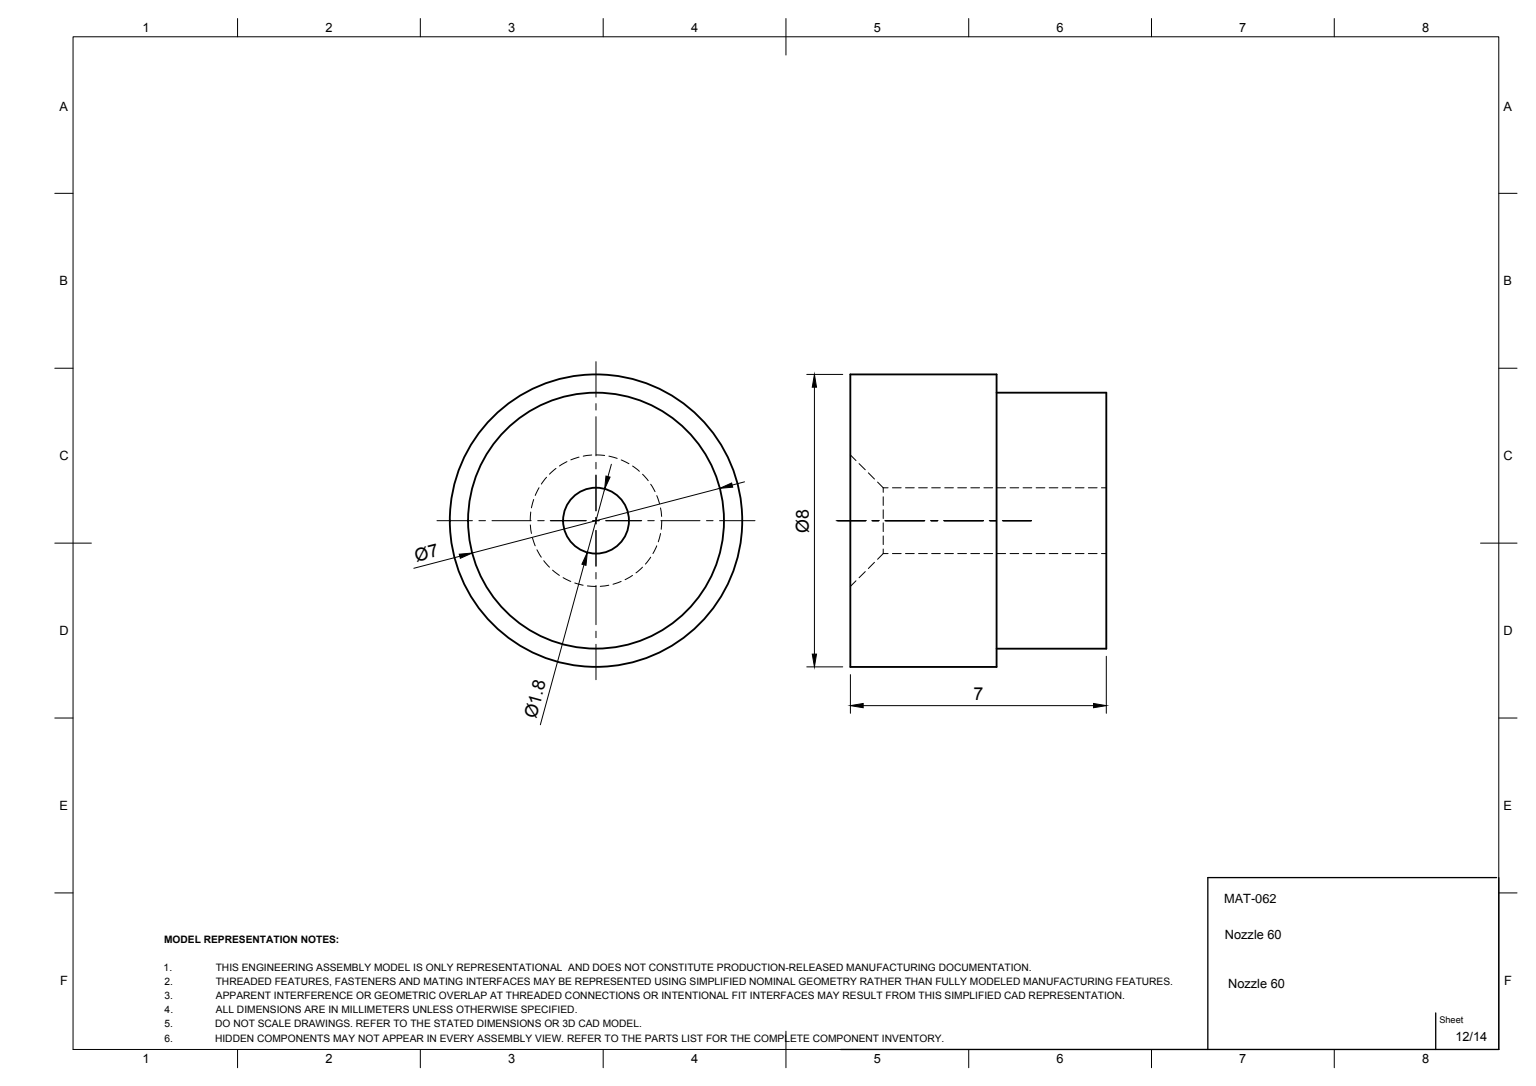
ISO-10303-21;
HEADER;
/* Generated by software containing ST-Developer
 * from STEP Tools, Inc. (www.steptools.com) 
 */

FILE_DESCRIPTION(
/* description */ (''),
/* implementation_level */ '2;1');

FILE_NAME(
/* name */ 'Nozzle 60.step',
/* time_stamp */ '2026-10-24T10:18:25-07:00',
/* author */ (''),
/* organization */ (''),
/* preprocessor_version */ 'ST-DEVELOPER v20.2',
/* originating_system */ 'Autodesk Translation Framework v15.15.0.0',
/* authorisation */ '');

FILE_SCHEMA (('AUTOMOTIVE_DESIGN { 1 0 10303 214 3 1 1 }'));
ENDSEC;

DATA;
#10=MECHANICAL_DESIGN_GEOMETRIC_PRESENTATION_REPRESENTATION('',(#260),#14125);
#194=CONICAL_SURFACE('',#6620,1.8,0.785398163397439);
#231=SHAPE_REPRESENTATION_RELATIONSHIP('SRR','None',#14205,#241);
#241=ADVANCED_BREP_SHAPE_REPRESENTATION('',(#273),#14119);
#260=STYLED_ITEM('',(#14263),#273);
#273=MANIFOLD_SOLID_BREP('Nozzle 60',#6141);
#554=CYLINDRICAL_SURFACE('',#6610,3.99999999999999);
#555=CYLINDRICAL_SURFACE('',#6617,0.899999999999993);
#556=CYLINDRICAL_SURFACE('',#6623,3.49999999999999);
#675=FACE_BOUND('',#1342,.T.);
#676=FACE_BOUND('',#1344,.T.);
#677=FACE_BOUND('',#1348,.T.);
#939=FACE_OUTER_BOUND('',#1340,.T.);
#940=FACE_OUTER_BOUND('',#1341,.T.);
#941=FACE_OUTER_BOUND('',#1343,.T.);
#942=FACE_OUTER_BOUND('',#1345,.T.);
#943=FACE_OUTER_BOUND('',#1346,.T.);
#944=FACE_OUTER_BOUND('',#1347,.T.);
#945=FACE_OUTER_BOUND('',#1349,.T.);
#1340=EDGE_LOOP('',(#4981,#4982,#4983,#4984));
#1341=EDGE_LOOP('',(#4985));
#1342=EDGE_LOOP('',(#4986));
#1343=EDGE_LOOP('',(#4987));
#1344=EDGE_LOOP('',(#4988));
#1345=EDGE_LOOP('',(#4989,#4990,#4991,#4992));
#1346=EDGE_LOOP('',(#4993,#4994,#4995,#4996));
#1347=EDGE_LOOP('',(#4997));
#1348=EDGE_LOOP('',(#4998));
#1349=EDGE_LOOP('',(#4999,#5000,#5001,#5002));
#1699=CIRCLE('',#6611,3.99999999999999);
#1700=CIRCLE('',#6612,3.99999999999999);
#1701=CIRCLE('',#6614,3.49999999999999);
#1702=CIRCLE('',#6616,1.8);
#1703=CIRCLE('',#6618,0.899999999999989);
#1704=CIRCLE('',#6619,0.899999999999988);
#1705=CIRCLE('',#6622,3.49999999999999);
#2038=LINE('',#12218,#2426);
#2039=LINE('',#12230,#2427);
#2040=LINE('',#12233,#2428);
#2041=LINE('',#12238,#2429);
#2426=VECTOR('',#7850,3.99999999999999);
#2427=VECTOR('',#7865,0.899999999999994);
#2428=VECTOR('',#7870,1.8);
#2429=VECTOR('',#7877,3.49999999999999);
#2916=VERTEX_POINT('',#12215);
#2917=VERTEX_POINT('',#12217);
#2918=VERTEX_POINT('',#12221);
#2919=VERTEX_POINT('',#12224);
#2920=VERTEX_POINT('',#12227);
#2921=VERTEX_POINT('',#12229);
#2922=VERTEX_POINT('',#12235);
#3638=EDGE_CURVE('',#2916,#2916,#1699,.T.);
#3639=EDGE_CURVE('',#2916,#2917,#2038,.T.);
#3640=EDGE_CURVE('',#2917,#2917,#1700,.T.);
#3641=EDGE_CURVE('',#2918,#2918,#1701,.T.);
#3642=EDGE_CURVE('',#2919,#2919,#1702,.T.);
#3643=EDGE_CURVE('',#2920,#2920,#1703,.T.);
#3644=EDGE_CURVE('',#2920,#2921,#2039,.T.);
#3645=EDGE_CURVE('',#2921,#2921,#1704,.T.);
#3646=EDGE_CURVE('',#2921,#2919,#2040,.T.);
#3647=EDGE_CURVE('',#2922,#2922,#1705,.T.);
#3648=EDGE_CURVE('',#2918,#2922,#2041,.T.);
#4981=ORIENTED_EDGE('',*,*,#3638,.T.);
#4982=ORIENTED_EDGE('',*,*,#3639,.T.);
#4983=ORIENTED_EDGE('',*,*,#3640,.F.);
#4984=ORIENTED_EDGE('',*,*,#3639,.F.);
#4985=ORIENTED_EDGE('',*,*,#3640,.T.);
#4986=ORIENTED_EDGE('',*,*,#3641,.F.);
#4987=ORIENTED_EDGE('',*,*,#3638,.F.);
#4988=ORIENTED_EDGE('',*,*,#3642,.F.);
#4989=ORIENTED_EDGE('',*,*,#3643,.T.);
#4990=ORIENTED_EDGE('',*,*,#3644,.T.);
#4991=ORIENTED_EDGE('',*,*,#3645,.T.);
#4992=ORIENTED_EDGE('',*,*,#3644,.F.);
#4993=ORIENTED_EDGE('',*,*,#3645,.F.);
#4994=ORIENTED_EDGE('',*,*,#3646,.T.);
#4995=ORIENTED_EDGE('',*,*,#3642,.T.);
#4996=ORIENTED_EDGE('',*,*,#3646,.F.);
#4997=ORIENTED_EDGE('',*,*,#3647,.T.);
#4998=ORIENTED_EDGE('',*,*,#3643,.F.);
#4999=ORIENTED_EDGE('',*,*,#3641,.T.);
#5000=ORIENTED_EDGE('',*,*,#3648,.T.);
#5001=ORIENTED_EDGE('',*,*,#3647,.F.);
#5002=ORIENTED_EDGE('',*,*,#3648,.F.);
#5716=PLANE('',#6613);
#5717=PLANE('',#6615);
#5718=PLANE('',#6621);
#5988=ADVANCED_FACE('',(#939),#554,.T.);
#5989=ADVANCED_FACE('',(#940,#675),#5716,.T.);
#5990=ADVANCED_FACE('',(#941,#676),#5717,.F.);
#5991=ADVANCED_FACE('',(#942),#555,.F.);
#5992=ADVANCED_FACE('',(#943),#194,.F.);
#5993=ADVANCED_FACE('',(#944,#677),#5718,.T.);
#5994=ADVANCED_FACE('',(#945),#556,.T.);
#6141=CLOSED_SHELL('',(#5988,#5989,#5990,#5991,#5992,#5993,#5994));
#6609=AXIS2_PLACEMENT_3D('',#12213,#7844,#7845);
#6610=AXIS2_PLACEMENT_3D('',#12214,#7846,#7847);
#6611=AXIS2_PLACEMENT_3D('',#12216,#7848,#7849);
#6612=AXIS2_PLACEMENT_3D('',#12219,#7851,#7852);
#6613=AXIS2_PLACEMENT_3D('',#12220,#7853,#7854);
#6614=AXIS2_PLACEMENT_3D('',#12222,#7855,#7856);
#6615=AXIS2_PLACEMENT_3D('',#12223,#7857,#7858);
#6616=AXIS2_PLACEMENT_3D('',#12225,#7859,#7860);
#6617=AXIS2_PLACEMENT_3D('',#12226,#7861,#7862);
#6618=AXIS2_PLACEMENT_3D('',#12228,#7863,#7864);
#6619=AXIS2_PLACEMENT_3D('',#12231,#7866,#7867);
#6620=AXIS2_PLACEMENT_3D('',#12232,#7868,#7869);
#6621=AXIS2_PLACEMENT_3D('',#12234,#7871,#7872);
#6622=AXIS2_PLACEMENT_3D('',#12236,#7873,#7874);
#6623=AXIS2_PLACEMENT_3D('',#12237,#7875,#7876);
#7844=DIRECTION('axis',(0.,0.,1.));
#7845=DIRECTION('refdir',(1.,0.,0.));
#7846=DIRECTION('center_axis',(-0.433012701892223,0.866025403784436,-0.250000000000002));
#7847=DIRECTION('ref_axis',(-0.894427190999914,-0.447213595499962,0.));
#7848=DIRECTION('center_axis',(0.433012701892223,-0.866025403784436,0.250000000000002));
#7849=DIRECTION('ref_axis',(0.894427190999914,0.447213595499962,0.));
#7850=DIRECTION('',(0.433012701892223,-0.866025403784436,0.250000000000002));
#7851=DIRECTION('center_axis',(0.433012701892223,-0.866025403784436,0.250000000000002));
#7852=DIRECTION('ref_axis',(0.894427190999914,0.447213595499962,0.));
#7853=DIRECTION('center_axis',(0.433012701892223,-0.866025403784436,0.250000000000002));
#7854=DIRECTION('ref_axis',(0.5,0.,-0.866025403784439));
#7855=DIRECTION('center_axis',(0.433012701892223,-0.866025403784437,0.250000000000002));
#7856=DIRECTION('ref_axis',(0.894427190999914,0.447213595499962,0.));
#7857=DIRECTION('center_axis',(0.433012701892223,-0.866025403784436,0.250000000000002));
#7858=DIRECTION('ref_axis',(0.5,0.,-0.866025403784439));
#7859=DIRECTION('center_axis',(-0.433012701892223,0.866025403784436,-0.250000000000002));
#7860=DIRECTION('ref_axis',(-0.894427190999914,-0.447213595499962,0.));
#7861=DIRECTION('center_axis',(-0.433012701892223,0.866025403784436,-0.250000000000002));
#7862=DIRECTION('ref_axis',(-0.894427190999914,-0.447213595499962,0.));
#7863=DIRECTION('center_axis',(0.433012701892223,-0.866025403784437,0.250000000000002));
#7864=DIRECTION('ref_axis',(0.894427190999914,0.447213595499962,0.));
#7865=DIRECTION('',(-0.433012701892223,0.866025403784436,-0.250000000000002));
#7866=DIRECTION('center_axis',(-0.433012701892223,0.866025403784436,-0.250000000000002));
#7867=DIRECTION('ref_axis',(-0.894427190999914,-0.447213595499962,0.));
#7868=DIRECTION('center_axis',(-0.433012701892223,0.866025403784436,-0.250000000000002));
#7869=DIRECTION('ref_axis',(-0.894427190999914,-0.447213595499962,0.));
#7870=DIRECTION('',(0.326269314185767,0.928600201712636,-0.17677669529664));
#7871=DIRECTION('center_axis',(0.433012701892223,-0.866025403784437,0.250000000000002));
#7872=DIRECTION('ref_axis',(0.5,0.,-0.866025403784439));
#7873=DIRECTION('center_axis',(0.433012701892223,-0.866025403784437,0.250000000000002));
#7874=DIRECTION('ref_axis',(0.894427190999914,0.447213595499962,0.));
#7875=DIRECTION('center_axis',(-0.433012701892223,0.866025403784436,-0.250000000000002));
#7876=DIRECTION('ref_axis',(-0.894427190999914,-0.447213595499962,0.));
#7877=DIRECTION('',(0.433012701892223,-0.866025403784436,0.250000000000002));
#12213=CARTESIAN_POINT('',(0.,0.,0.));
#12214=CARTESIAN_POINT('Origin',(-102.211351574804,130.535898384862,-71.0117513459462));
#12215=CARTESIAN_POINT('',(-100.365693618373,135.788854382,-72.0117513459462));
#12216=CARTESIAN_POINT('Origin',(-103.943402382373,134.,-72.0117513459462));
#12217=CARTESIAN_POINT('',(-98.6336428108046,132.324752766862,-71.0117513459462));
#12218=CARTESIAN_POINT('',(-98.6336428108046,132.324752766862,-71.0117513459462));
#12219=CARTESIAN_POINT('Origin',(-102.211351574804,130.535898384862,-71.0117513459462));
#12220=CARTESIAN_POINT('Origin',(-102.211351574804,130.535898384862,-71.0117513459462));
#12221=CARTESIAN_POINT('',(-99.0808564063046,132.101145969112,-71.0117513459462));
#12222=CARTESIAN_POINT('Origin',(-102.211351574804,130.535898384862,-71.0117513459462));
#12223=CARTESIAN_POINT('Origin',(-103.943402382373,134.,-72.0117513459462));
#12224=CARTESIAN_POINT('',(-102.333433438573,134.8049844719,-72.0117513459462));
#12225=CARTESIAN_POINT('Origin',(-103.943402382373,134.,-72.0117513459462));
#12226=CARTESIAN_POINT('Origin',(-103.943402382373,134.,-72.0117513459462));
#12227=CARTESIAN_POINT('',(-100.107328997228,128.340314409459,-70.2617513459462));
#12228=CARTESIAN_POINT('Origin',(-100.912313469128,127.937822173509,-70.2617513459462));
#12229=CARTESIAN_POINT('',(-102.74870647877,133.623069372544,-71.7867513459462));
#12230=CARTESIAN_POINT('',(-103.138417910473,134.40249223595,-72.0117513459462));
#12231=CARTESIAN_POINT('Origin',(-103.55369095067,133.220577136594,-71.7867513459462));
#12232=CARTESIAN_POINT('Origin',(-103.943402382373,134.,-72.0117513459462));
#12233=CARTESIAN_POINT('',(-102.333433438573,134.8049844719,-72.0117513459462));
#12234=CARTESIAN_POINT('Origin',(-100.912313469128,127.937822173509,-70.2617513459462));
#12235=CARTESIAN_POINT('',(-97.7818183006279,129.503069757759,-70.2617513459462));
#12236=CARTESIAN_POINT('Origin',(-100.912313469128,127.937822173509,-70.2617513459462));
#12237=CARTESIAN_POINT('Origin',(-100.912313469128,127.937822173509,-70.2617513459462));
#12238=CARTESIAN_POINT('',(-97.7818183006279,129.503069757759,-70.2617513459462));
#14106=UNCERTAINTY_MEASURE_WITH_UNIT(LENGTH_MEASURE(0.01),#14126,
'DISTANCE_ACCURACY_VALUE',
'Maximum model space distance between geometric entities at asserted c
onnectivities');
#14112=UNCERTAINTY_MEASURE_WITH_UNIT(LENGTH_MEASURE(0.01),#14126,
'DISTANCE_ACCURACY_VALUE',
'Maximum model space distance between geometric entities at asserted c
onnectivities');
#14119=(
GEOMETRIC_REPRESENTATION_CONTEXT(3)
GLOBAL_UNCERTAINTY_ASSIGNED_CONTEXT((#14106))
GLOBAL_UNIT_ASSIGNED_CONTEXT((#14126,#14128,#14129))
REPRESENTATION_CONTEXT('','3D')
);
#14125=(
GEOMETRIC_REPRESENTATION_CONTEXT(3)
GLOBAL_UNCERTAINTY_ASSIGNED_CONTEXT((#14112))
GLOBAL_UNIT_ASSIGNED_CONTEXT((#14126,#14128,#14129))
REPRESENTATION_CONTEXT('','3D')
);
#14126=(
LENGTH_UNIT()
NAMED_UNIT(*)
SI_UNIT(.MILLI.,.METRE.)
);
#14128=(
NAMED_UNIT(*)
PLANE_ANGLE_UNIT()
SI_UNIT($,.RADIAN.)
);
#14129=(
NAMED_UNIT(*)
SI_UNIT($,.STERADIAN.)
SOLID_ANGLE_UNIT()
);
#14136=SHAPE_DEFINITION_REPRESENTATION(#14148,#14205);
#14148=PRODUCT_DEFINITION_SHAPE('',$,#14218);
#14205=SHAPE_REPRESENTATION('',(#6609),#14119);
#14211=PRODUCT_DEFINITION_CONTEXT('part definition',#14249,'design');
#14218=PRODUCT_DEFINITION('Nozzle 60','Nozzle 60',#14230,#14211);
#14230=PRODUCT_DEFINITION_FORMATION('',$,#14257);
#14249=APPLICATION_CONTEXT(
'Core Data for Automotive Mechanical Design Process');
#14250=PRODUCT_CONTEXT('part definition',#14249,'mechanical');
#14257=PRODUCT('Nozzle 60','Nozzle 60',$,(#14250));
#14263=PRESENTATION_STYLE_ASSIGNMENT((#14265));
#14265=SURFACE_STYLE_USAGE(.BOTH.,#14267);
#14267=SURFACE_SIDE_STYLE('',(#14269));
#14269=SURFACE_STYLE_FILL_AREA(#14271);
#14271=FILL_AREA_STYLE('Steel - Satin',(#14273));
#14273=FILL_AREA_STYLE_COLOUR('Steel - Satin',#14275);
#14275=COLOUR_RGB('Steel - Satin',0.627450980392157,0.627450980392157,0.627450980392157);
ENDSEC;
END-ISO-10303-21;
